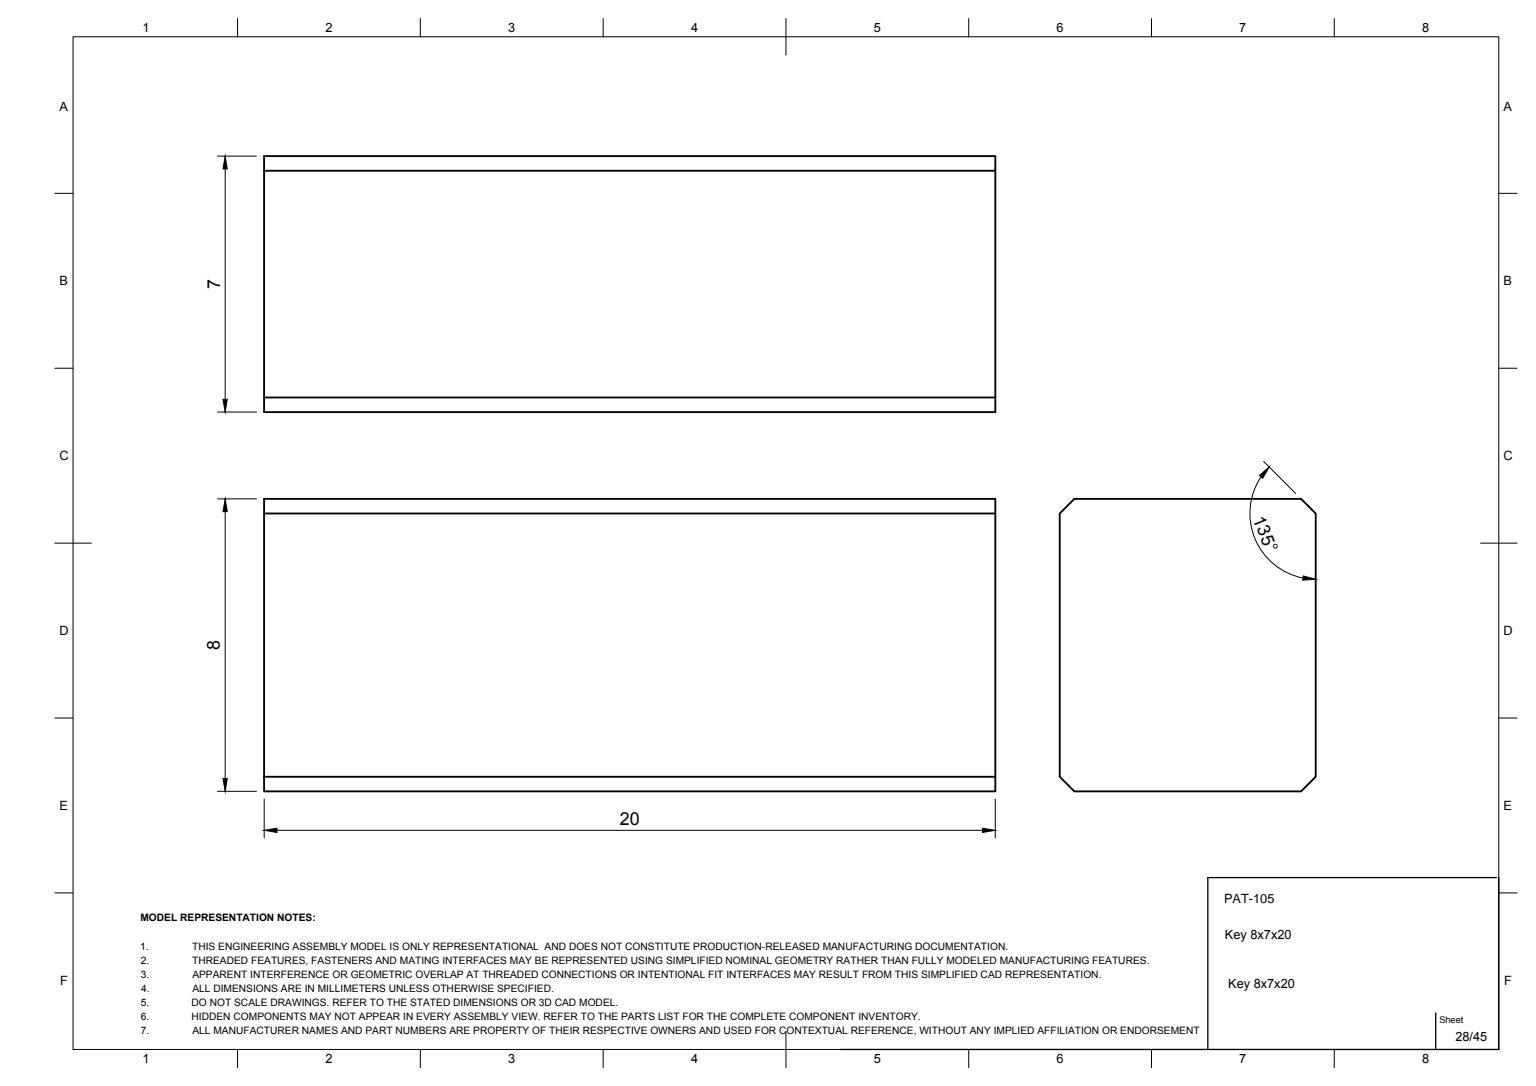
ISO-10303-21;
HEADER;
/* Generated by software containing ST-Developer
 * from STEP Tools, Inc. (www.steptools.com) 
 */

FILE_DESCRIPTION(
/* description */ ('Torque wrench calibration arm'),
/* implementation_level */ '2;1');

FILE_NAME(
/* name */ 'Key 8x7x20.step',
/* time_stamp */ '2026-10-28T03:24:52-07:00',
/* author */ (''),
/* organization */ (''),
/* preprocessor_version */ 'ST-DEVELOPER v20.2',
/* originating_system */ 'Autodesk Translation Framework v15.17.0.0',
/* authorisation */ '');

FILE_SCHEMA (('AUTOMOTIVE_DESIGN { 1 0 10303 214 3 1 1 }'));
ENDSEC;

DATA;
#10=MECHANICAL_DESIGN_GEOMETRIC_PRESENTATION_REPRESENTATION('',(#456),#12783);
#373=SHAPE_REPRESENTATION_RELATIONSHIP('SRR','None',#12956,#410);
#410=ADVANCED_BREP_SHAPE_REPRESENTATION('',(#508),#12765);
#456=STYLED_ITEM('',(#13212),#508);
#508=MANIFOLD_SOLID_BREP('Body1',#6527);
#802=PLANE('',#7510);
#803=PLANE('',#7511);
#804=PLANE('',#7512);
#805=PLANE('',#7513);
#806=PLANE('',#7514);
#807=PLANE('',#7515);
#808=PLANE('',#7516);
#809=PLANE('',#7517);
#810=PLANE('',#7518);
#811=PLANE('',#7519);
#1137=FACE_OUTER_BOUND('',#1622,.T.);
#1138=FACE_OUTER_BOUND('',#1623,.T.);
#1139=FACE_OUTER_BOUND('',#1624,.T.);
#1140=FACE_OUTER_BOUND('',#1625,.T.);
#1141=FACE_OUTER_BOUND('',#1626,.T.);
#1142=FACE_OUTER_BOUND('',#1627,.T.);
#1143=FACE_OUTER_BOUND('',#1628,.T.);
#1144=FACE_OUTER_BOUND('',#1629,.T.);
#1145=FACE_OUTER_BOUND('',#1630,.T.);
#1146=FACE_OUTER_BOUND('',#1631,.T.);
#1622=EDGE_LOOP('',(#5461,#5462,#5463,#5464,#5465,#5466,#5467,#5468));
#1623=EDGE_LOOP('',(#5469,#5470,#5471,#5472));
#1624=EDGE_LOOP('',(#5473,#5474,#5475,#5476));
#1625=EDGE_LOOP('',(#5477,#5478,#5479,#5480));
#1626=EDGE_LOOP('',(#5481,#5482,#5483,#5484));
#1627=EDGE_LOOP('',(#5485,#5486,#5487,#5488,#5489,#5490,#5491,#5492));
#1628=EDGE_LOOP('',(#5493,#5494,#5495,#5496));
#1629=EDGE_LOOP('',(#5497,#5498,#5499,#5500));
#1630=EDGE_LOOP('',(#5501,#5502,#5503,#5504));
#1631=EDGE_LOOP('',(#5505,#5506,#5507,#5508));
#2075=LINE('',#11734,#2490);
#2076=LINE('',#11736,#2491);
#2077=LINE('',#11738,#2492);
#2078=LINE('',#11740,#2493);
#2079=LINE('',#11742,#2494);
#2080=LINE('',#11744,#2495);
#2081=LINE('',#11746,#2496);
#2082=LINE('',#11747,#2497);
#2083=LINE('',#11750,#2498);
#2084=LINE('',#11752,#2499);
#2085=LINE('',#11753,#2500);
#2086=LINE('',#11756,#2501);
#2087=LINE('',#11757,#2502);
#2088=LINE('',#11760,#2503);
#2089=LINE('',#11761,#2504);
#2090=LINE('',#11764,#2505);
#2091=LINE('',#11765,#2506);
#2092=LINE('',#11768,#2507);
#2093=LINE('',#11770,#2508);
#2094=LINE('',#11772,#2509);
#2095=LINE('',#11773,#2510);
#2096=LINE('',#11775,#2511);
#2097=LINE('',#11777,#2512);
#2098=LINE('',#11779,#2513);
#2490=VECTOR('',#9201,1.);
#2491=VECTOR('',#9202,1.);
#2492=VECTOR('',#9203,1.);
#2493=VECTOR('',#9204,1.);
#2494=VECTOR('',#9205,1.);
#2495=VECTOR('',#9206,1.);
#2496=VECTOR('',#9207,1.);
#2497=VECTOR('',#9208,1.);
#2498=VECTOR('',#9211,1.);
#2499=VECTOR('',#9212,1.);
#2500=VECTOR('',#9213,1.);
#2501=VECTOR('',#9216,1.);
#2502=VECTOR('',#9217,1.);
#2503=VECTOR('',#9220,1.);
#2504=VECTOR('',#9221,1.);
#2505=VECTOR('',#9224,1.);
#2506=VECTOR('',#9225,1.);
#2507=VECTOR('',#9228,1.);
#2508=VECTOR('',#9229,1.);
#2509=VECTOR('',#9230,1.);
#2510=VECTOR('',#9231,1.);
#2511=VECTOR('',#9234,1.);
#2512=VECTOR('',#9237,1.);
#2513=VECTOR('',#9240,1.);
#3350=VERTEX_POINT('',#11732);
#3351=VERTEX_POINT('',#11733);
#3352=VERTEX_POINT('',#11735);
#3353=VERTEX_POINT('',#11737);
#3354=VERTEX_POINT('',#11739);
#3355=VERTEX_POINT('',#11741);
#3356=VERTEX_POINT('',#11743);
#3357=VERTEX_POINT('',#11745);
#3358=VERTEX_POINT('',#11749);
#3359=VERTEX_POINT('',#11751);
#3360=VERTEX_POINT('',#11755);
#3361=VERTEX_POINT('',#11759);
#3362=VERTEX_POINT('',#11763);
#3363=VERTEX_POINT('',#11767);
#3364=VERTEX_POINT('',#11769);
#3365=VERTEX_POINT('',#11771);
#4088=EDGE_CURVE('',#3350,#3351,#2075,.T.);
#4089=EDGE_CURVE('',#3352,#3350,#2076,.T.);
#4090=EDGE_CURVE('',#3353,#3352,#2077,.T.);
#4091=EDGE_CURVE('',#3354,#3353,#2078,.T.);
#4092=EDGE_CURVE('',#3355,#3354,#2079,.T.);
#4093=EDGE_CURVE('',#3356,#3355,#2080,.T.);
#4094=EDGE_CURVE('',#3357,#3356,#2081,.T.);
#4095=EDGE_CURVE('',#3351,#3357,#2082,.T.);
#4096=EDGE_CURVE('',#3354,#3358,#2083,.T.);
#4097=EDGE_CURVE('',#3358,#3359,#2084,.T.);
#4098=EDGE_CURVE('',#3359,#3355,#2085,.T.);
#4099=EDGE_CURVE('',#3360,#3353,#2086,.T.);
#4100=EDGE_CURVE('',#3360,#3358,#2087,.T.);
#4101=EDGE_CURVE('',#3352,#3361,#2088,.T.);
#4102=EDGE_CURVE('',#3361,#3360,#2089,.T.);
#4103=EDGE_CURVE('',#3362,#3350,#2090,.T.);
#4104=EDGE_CURVE('',#3362,#3361,#2091,.T.);
#4105=EDGE_CURVE('',#3363,#3362,#2092,.T.);
#4106=EDGE_CURVE('',#3364,#3363,#2093,.T.);
#4107=EDGE_CURVE('',#3365,#3364,#2094,.T.);
#4108=EDGE_CURVE('',#3359,#3365,#2095,.T.);
#4109=EDGE_CURVE('',#3351,#3363,#2096,.T.);
#4110=EDGE_CURVE('',#3364,#3357,#2097,.T.);
#4111=EDGE_CURVE('',#3356,#3365,#2098,.T.);
#5461=ORIENTED_EDGE('',*,*,#4088,.F.);
#5462=ORIENTED_EDGE('',*,*,#4089,.F.);
#5463=ORIENTED_EDGE('',*,*,#4090,.F.);
#5464=ORIENTED_EDGE('',*,*,#4091,.F.);
#5465=ORIENTED_EDGE('',*,*,#4092,.F.);
#5466=ORIENTED_EDGE('',*,*,#4093,.F.);
#5467=ORIENTED_EDGE('',*,*,#4094,.F.);
#5468=ORIENTED_EDGE('',*,*,#4095,.F.);
#5469=ORIENTED_EDGE('',*,*,#4092,.T.);
#5470=ORIENTED_EDGE('',*,*,#4096,.T.);
#5471=ORIENTED_EDGE('',*,*,#4097,.T.);
#5472=ORIENTED_EDGE('',*,*,#4098,.T.);
#5473=ORIENTED_EDGE('',*,*,#4091,.T.);
#5474=ORIENTED_EDGE('',*,*,#4099,.F.);
#5475=ORIENTED_EDGE('',*,*,#4100,.T.);
#5476=ORIENTED_EDGE('',*,*,#4096,.F.);
#5477=ORIENTED_EDGE('',*,*,#4090,.T.);
#5478=ORIENTED_EDGE('',*,*,#4101,.T.);
#5479=ORIENTED_EDGE('',*,*,#4102,.T.);
#5480=ORIENTED_EDGE('',*,*,#4099,.T.);
#5481=ORIENTED_EDGE('',*,*,#4089,.T.);
#5482=ORIENTED_EDGE('',*,*,#4103,.F.);
#5483=ORIENTED_EDGE('',*,*,#4104,.T.);
#5484=ORIENTED_EDGE('',*,*,#4101,.F.);
#5485=ORIENTED_EDGE('',*,*,#4097,.F.);
#5486=ORIENTED_EDGE('',*,*,#4100,.F.);
#5487=ORIENTED_EDGE('',*,*,#4102,.F.);
#5488=ORIENTED_EDGE('',*,*,#4104,.F.);
#5489=ORIENTED_EDGE('',*,*,#4105,.F.);
#5490=ORIENTED_EDGE('',*,*,#4106,.F.);
#5491=ORIENTED_EDGE('',*,*,#4107,.F.);
#5492=ORIENTED_EDGE('',*,*,#4108,.F.);
#5493=ORIENTED_EDGE('',*,*,#4088,.T.);
#5494=ORIENTED_EDGE('',*,*,#4109,.T.);
#5495=ORIENTED_EDGE('',*,*,#4105,.T.);
#5496=ORIENTED_EDGE('',*,*,#4103,.T.);
#5497=ORIENTED_EDGE('',*,*,#4095,.T.);
#5498=ORIENTED_EDGE('',*,*,#4110,.F.);
#5499=ORIENTED_EDGE('',*,*,#4106,.T.);
#5500=ORIENTED_EDGE('',*,*,#4109,.F.);
#5501=ORIENTED_EDGE('',*,*,#4094,.T.);
#5502=ORIENTED_EDGE('',*,*,#4111,.T.);
#5503=ORIENTED_EDGE('',*,*,#4107,.T.);
#5504=ORIENTED_EDGE('',*,*,#4110,.T.);
#5505=ORIENTED_EDGE('',*,*,#4093,.T.);
#5506=ORIENTED_EDGE('',*,*,#4098,.F.);
#5507=ORIENTED_EDGE('',*,*,#4108,.T.);
#5508=ORIENTED_EDGE('',*,*,#4111,.F.);
#6362=ADVANCED_FACE('',(#1137),#802,.T.);
#6363=ADVANCED_FACE('',(#1138),#803,.T.);
#6364=ADVANCED_FACE('',(#1139),#804,.T.);
#6365=ADVANCED_FACE('',(#1140),#805,.T.);
#6366=ADVANCED_FACE('',(#1141),#806,.T.);
#6367=ADVANCED_FACE('',(#1142),#807,.F.);
#6368=ADVANCED_FACE('',(#1143),#808,.T.);
#6369=ADVANCED_FACE('',(#1144),#809,.T.);
#6370=ADVANCED_FACE('',(#1145),#810,.T.);
#6371=ADVANCED_FACE('',(#1146),#811,.F.);
#6527=CLOSED_SHELL('',(#6362,#6363,#6364,#6365,#6366,#6367,#6368,#6369,
#6370,#6371));
#7509=AXIS2_PLACEMENT_3D('',#11730,#9197,#9198);
#7510=AXIS2_PLACEMENT_3D('',#11731,#9199,#9200);
#7511=AXIS2_PLACEMENT_3D('',#11748,#9209,#9210);
#7512=AXIS2_PLACEMENT_3D('',#11754,#9214,#9215);
#7513=AXIS2_PLACEMENT_3D('',#11758,#9218,#9219);
#7514=AXIS2_PLACEMENT_3D('',#11762,#9222,#9223);
#7515=AXIS2_PLACEMENT_3D('',#11766,#9226,#9227);
#7516=AXIS2_PLACEMENT_3D('',#11774,#9232,#9233);
#7517=AXIS2_PLACEMENT_3D('',#11776,#9235,#9236);
#7518=AXIS2_PLACEMENT_3D('',#11778,#9238,#9239);
#7519=AXIS2_PLACEMENT_3D('',#11780,#9241,#9242);
#9197=DIRECTION('axis',(0.,0.,1.));
#9198=DIRECTION('refdir',(1.,0.,0.));
#9199=DIRECTION('center_axis',(1.,0.,0.));
#9200=DIRECTION('ref_axis',(0.,0.,-1.));
#9201=DIRECTION('',(0.,0.707106781186548,-0.707106781186548));
#9202=DIRECTION('',(0.,1.,0.));
#9203=DIRECTION('',(0.,0.707106781186548,0.707106781186548));
#9204=DIRECTION('',(0.,0.,1.));
#9205=DIRECTION('',(0.,-0.707106781186548,0.707106781186547));
#9206=DIRECTION('',(0.,-1.,0.));
#9207=DIRECTION('',(0.,-0.707106781186548,-0.707106781186547));
#9208=DIRECTION('',(0.,0.,-1.));
#9209=DIRECTION('center_axis',(0.,-0.707106781186547,-0.707106781186548));
#9210=DIRECTION('ref_axis',(-1.,0.,0.));
#9211=DIRECTION('',(-1.,0.,0.));
#9212=DIRECTION('',(0.,0.707106781186548,-0.707106781186547));
#9213=DIRECTION('',(1.,0.,0.));
#9214=DIRECTION('center_axis',(0.,-1.,0.));
#9215=DIRECTION('ref_axis',(1.,0.,0.));
#9216=DIRECTION('',(1.,0.,0.));
#9217=DIRECTION('',(0.,0.,-1.));
#9218=DIRECTION('center_axis',(0.,-0.707106781186548,0.707106781186548));
#9219=DIRECTION('ref_axis',(1.,0.,0.));
#9220=DIRECTION('',(-1.,0.,0.));
#9221=DIRECTION('',(0.,-0.707106781186548,-0.707106781186548));
#9222=DIRECTION('center_axis',(0.,0.,1.));
#9223=DIRECTION('ref_axis',(1.,0.,0.));
#9224=DIRECTION('',(1.,0.,0.));
#9225=DIRECTION('',(0.,-1.,0.));
#9226=DIRECTION('center_axis',(1.,0.,0.));
#9227=DIRECTION('ref_axis',(0.,0.,-1.));
#9228=DIRECTION('',(0.,-0.707106781186548,0.707106781186548));
#9229=DIRECTION('',(0.,0.,1.));
#9230=DIRECTION('',(0.,0.707106781186548,0.707106781186547));
#9231=DIRECTION('',(0.,1.,0.));
#9232=DIRECTION('center_axis',(0.,0.707106781186548,0.707106781186548));
#9233=DIRECTION('ref_axis',(1.,0.,0.));
#9234=DIRECTION('',(-1.,0.,0.));
#9235=DIRECTION('center_axis',(0.,1.,0.));
#9236=DIRECTION('ref_axis',(-1.,0.,0.));
#9237=DIRECTION('',(1.,0.,0.));
#9238=DIRECTION('center_axis',(0.,0.707106781186547,-0.707106781186548));
#9239=DIRECTION('ref_axis',(-1.,0.,0.));
#9240=DIRECTION('',(-1.,0.,0.));
#9241=DIRECTION('center_axis',(0.,0.,1.));
#9242=DIRECTION('ref_axis',(1.,0.,0.));
#11730=CARTESIAN_POINT('',(0.,0.,0.));
#11731=CARTESIAN_POINT('Origin',(1.,0.,0.4));
#11732=CARTESIAN_POINT('',(1.,0.36,0.7));
#11733=CARTESIAN_POINT('',(1.,0.4,0.66));
#11734=CARTESIAN_POINT('',(1.,0.355,0.705));
#11735=CARTESIAN_POINT('',(1.,-0.36,0.7));
#11736=CARTESIAN_POINT('',(1.,0.,0.7));
#11737=CARTESIAN_POINT('',(1.,-0.4,0.66));
#11738=CARTESIAN_POINT('',(1.,-0.355,0.705));
#11739=CARTESIAN_POINT('',(1.,-0.4,0.04));
#11740=CARTESIAN_POINT('',(1.,-0.4,0.2));
#11741=CARTESIAN_POINT('',(1.,-0.36,0.));
#11742=CARTESIAN_POINT('',(1.,-0.38,0.0199999999999999));
#11743=CARTESIAN_POINT('',(1.,0.36,0.));
#11744=CARTESIAN_POINT('',(1.,0.,0.));
#11745=CARTESIAN_POINT('',(1.,0.4,0.04));
#11746=CARTESIAN_POINT('',(1.,0.38,0.0199999999999999));
#11747=CARTESIAN_POINT('',(1.,0.4,0.2));
#11748=CARTESIAN_POINT('Origin',(-0.8,-0.38,0.02));
#11749=CARTESIAN_POINT('',(-1.,-0.4,0.04));
#11750=CARTESIAN_POINT('',(-0.8,-0.4,0.04));
#11751=CARTESIAN_POINT('',(-1.,-0.36,0.));
#11752=CARTESIAN_POINT('',(-1.,-0.38,0.0199999999999999));
#11753=CARTESIAN_POINT('',(-0.8,-0.36,0.));
#11754=CARTESIAN_POINT('Origin',(-1.6,-0.4,0.));
#11755=CARTESIAN_POINT('',(-1.,-0.4,0.66));
#11756=CARTESIAN_POINT('',(-0.8,-0.4,0.66));
#11757=CARTESIAN_POINT('',(-1.,-0.4,0.2));
#11758=CARTESIAN_POINT('Origin',(-0.8,-0.38,0.68));
#11759=CARTESIAN_POINT('',(-1.,-0.36,0.7));
#11760=CARTESIAN_POINT('',(-0.8,-0.36,0.7));
#11761=CARTESIAN_POINT('',(-1.,-0.355,0.705));
#11762=CARTESIAN_POINT('Origin',(0.,0.,0.7));
#11763=CARTESIAN_POINT('',(-1.,0.36,0.7));
#11764=CARTESIAN_POINT('',(0.8,0.36,0.7));
#11765=CARTESIAN_POINT('',(-1.,0.,0.7));
#11766=CARTESIAN_POINT('Origin',(-1.,0.,0.4));
#11767=CARTESIAN_POINT('',(-1.,0.4,0.66));
#11768=CARTESIAN_POINT('',(-1.,0.355,0.705));
#11769=CARTESIAN_POINT('',(-1.,0.4,0.04));
#11770=CARTESIAN_POINT('',(-1.,0.4,0.2));
#11771=CARTESIAN_POINT('',(-1.,0.36,0.));
#11772=CARTESIAN_POINT('',(-1.,0.38,0.0199999999999999));
#11773=CARTESIAN_POINT('',(-1.,0.,0.));
#11774=CARTESIAN_POINT('Origin',(0.8,0.38,0.68));
#11775=CARTESIAN_POINT('',(0.8,0.4,0.66));
#11776=CARTESIAN_POINT('Origin',(1.6,0.4,0.));
#11777=CARTESIAN_POINT('',(0.8,0.4,0.04));
#11778=CARTESIAN_POINT('Origin',(0.8,0.38,0.02));
#11779=CARTESIAN_POINT('',(0.8,0.36,0.));
#11780=CARTESIAN_POINT('Origin',(0.,0.,0.));
#12721=UNCERTAINTY_MEASURE_WITH_UNIT(LENGTH_MEASURE(0.001),#12784,
'DISTANCE_ACCURACY_VALUE',
'Maximum model space distance between geometric entities at asserted c
onnectivities');
#12739=UNCERTAINTY_MEASURE_WITH_UNIT(LENGTH_MEASURE(0.001),#12784,
'DISTANCE_ACCURACY_VALUE',
'Maximum model space distance between geometric entities at asserted c
onnectivities');
#12765=(
GEOMETRIC_REPRESENTATION_CONTEXT(3)
GLOBAL_UNCERTAINTY_ASSIGNED_CONTEXT((#12721))
GLOBAL_UNIT_ASSIGNED_CONTEXT((#12784,#12786,#12787))
REPRESENTATION_CONTEXT('','3D')
);
#12783=(
GEOMETRIC_REPRESENTATION_CONTEXT(3)
GLOBAL_UNCERTAINTY_ASSIGNED_CONTEXT((#12739))
GLOBAL_UNIT_ASSIGNED_CONTEXT((#12784,#12786,#12787))
REPRESENTATION_CONTEXT('','3D')
);
#12784=(
LENGTH_UNIT()
NAMED_UNIT(*)
SI_UNIT(.CENTI.,.METRE.)
);
#12786=(
NAMED_UNIT(*)
PLANE_ANGLE_UNIT()
SI_UNIT($,.RADIAN.)
);
#12787=(
NAMED_UNIT(*)
SI_UNIT($,.STERADIAN.)
SOLID_ANGLE_UNIT()
);
#12813=SHAPE_DEFINITION_REPRESENTATION(#12882,#12956);
#12882=PRODUCT_DEFINITION_SHAPE('',$,#13000);
#12956=SHAPE_REPRESENTATION('',(#7509),#12765);
#12974=PRODUCT_DEFINITION_CONTEXT('part definition',#13105,'design');
#13000=PRODUCT_DEFINITION('Key 8x7x20','Key 8x7x20',#13043,#12974);
#13043=PRODUCT_DEFINITION_FORMATION('',$,#13132);
#13105=APPLICATION_CONTEXT(
'Core Data for Automotive Mechanical Design Process');
#13106=PRODUCT_CONTEXT('part definition',#13105,'mechanical');
#13132=PRODUCT('Key 8x7x20','Key 8x7x20','Key 8x7x20',(#13106));
#13206=COLOUR_RGB('Grey',0.48,0.52,0.57);
#13207=FILL_AREA_STYLE_COLOUR('',#13206);
#13208=FILL_AREA_STYLE('',(#13207));
#13209=SURFACE_STYLE_FILL_AREA(#13208);
#13210=SURFACE_SIDE_STYLE('',(#13209));
#13211=SURFACE_STYLE_USAGE(.BOTH.,#13210);
#13212=PRESENTATION_STYLE_ASSIGNMENT((#13211));
ENDSEC;
END-ISO-10303-21;
